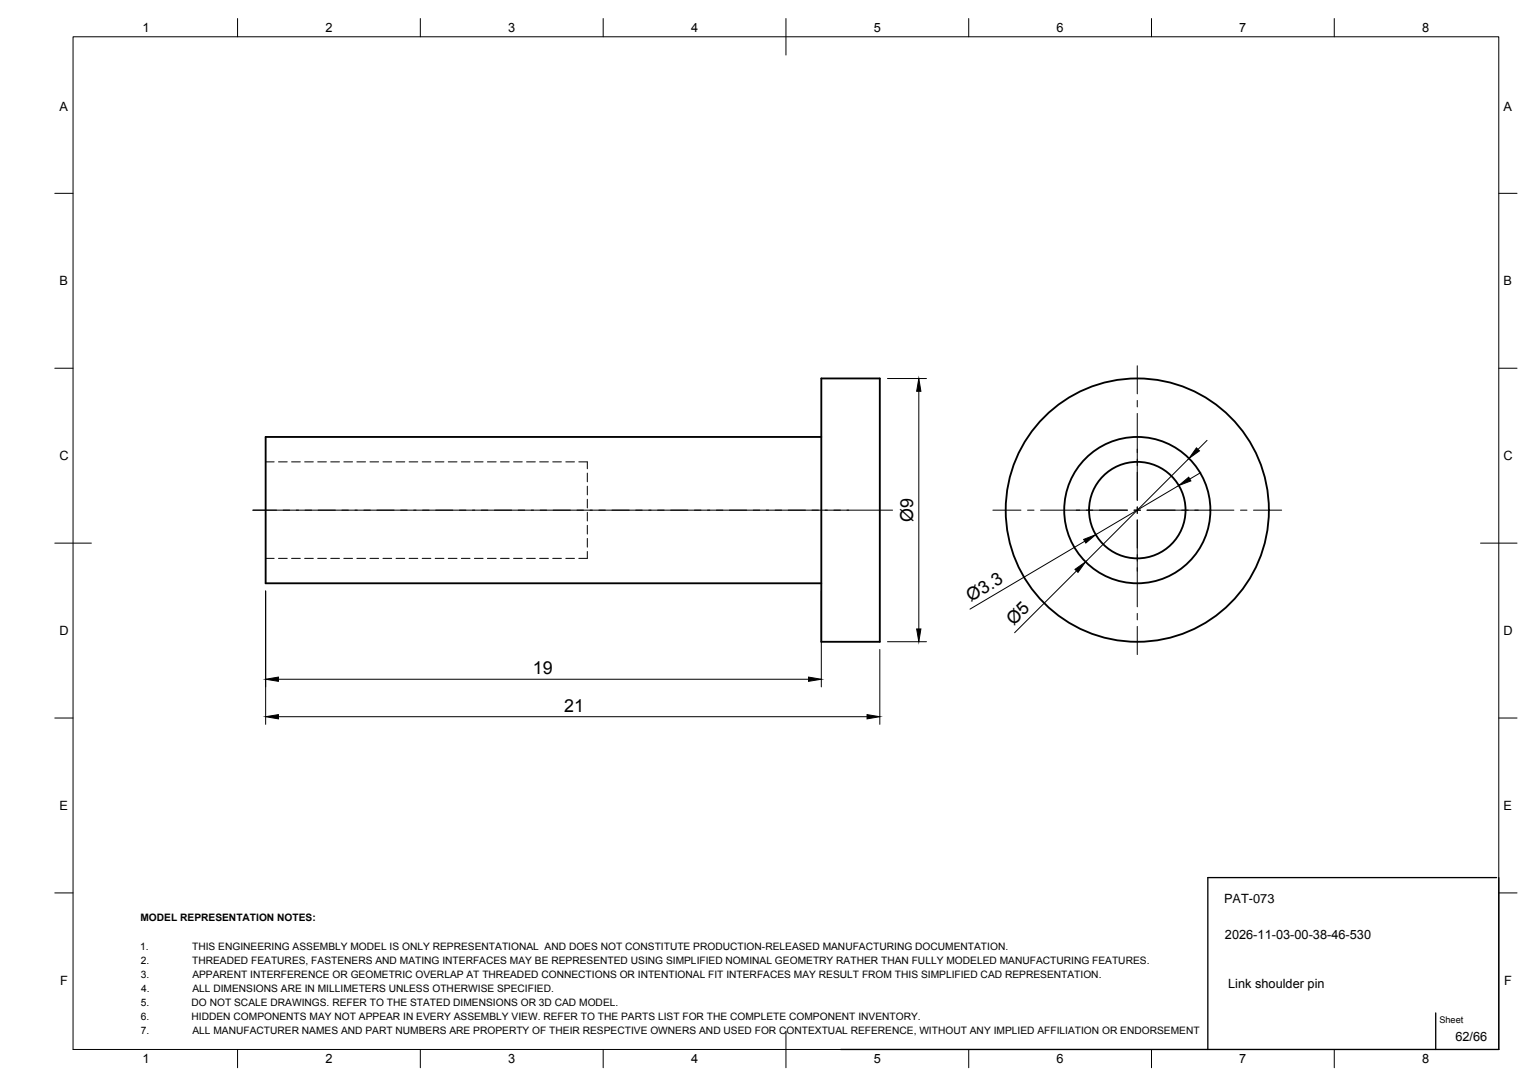
ISO-10303-21;
HEADER;
/* Generated by software containing ST-Developer
 * from STEP Tools, Inc. (www.steptools.com) 
 */

FILE_DESCRIPTION(
/* description */ ('Manual piston pump'),
/* implementation_level */ '2;1');

FILE_NAME(
/* name */ 'Link shoulder pin.step',
/* time_stamp */ '2026-11-02T16:54:23-08:00',
/* author */ (''),
/* organization */ (''),
/* preprocessor_version */ 'ST-DEVELOPER v20.2',
/* originating_system */ 'Autodesk Translation Framework v15.17.0.0',
/* authorisation */ '');

FILE_SCHEMA (('AUTOMOTIVE_DESIGN { 1 0 10303 214 3 1 1 }'));
ENDSEC;

DATA;
#10=MECHANICAL_DESIGN_GEOMETRIC_PRESENTATION_REPRESENTATION('',(#754),#19043);
#619=SHAPE_REPRESENTATION_RELATIONSHIP('SRR','None',#19369,#682);
#682=ADVANCED_BREP_SHAPE_REPRESENTATION('',(#822),#19036);
#754=STYLED_ITEM('',(#19661),#822);
#822=MANIFOLD_SOLID_BREP('Body1',#9542);
#1035=FACE_BOUND('',#2610,.T.);
#1036=FACE_BOUND('',#2615,.T.);
#1277=CYLINDRICAL_SURFACE('',#11382,0.164999999999999);
#1278=CYLINDRICAL_SURFACE('',#11389,0.449999999999999);
#1279=CYLINDRICAL_SURFACE('',#11392,0.25);
#1824=FACE_OUTER_BOUND('',#2607,.T.);
#1825=FACE_OUTER_BOUND('',#2608,.T.);
#1826=FACE_OUTER_BOUND('',#2609,.T.);
#1827=FACE_OUTER_BOUND('',#2611,.T.);
#1828=FACE_OUTER_BOUND('',#2612,.T.);
#1829=FACE_OUTER_BOUND('',#2613,.T.);
#1830=FACE_OUTER_BOUND('',#2614,.T.);
#2607=EDGE_LOOP('',(#8423,#8424,#8425,#8426));
#2608=EDGE_LOOP('',(#8427));
#2609=EDGE_LOOP('',(#8428));
#2610=EDGE_LOOP('',(#8429));
#2611=EDGE_LOOP('',(#8430,#8431,#8432,#8433));
#2612=EDGE_LOOP('',(#8434));
#2613=EDGE_LOOP('',(#8435,#8436,#8437,#8438));
#2614=EDGE_LOOP('',(#8439));
#2615=EDGE_LOOP('',(#8440));
#3114=CIRCLE('',#11383,0.164999999999999);
#3115=CIRCLE('',#11384,0.164999999999999);
#3116=CIRCLE('',#11387,0.449999999999999);
#3117=CIRCLE('',#11388,0.25);
#3118=CIRCLE('',#11390,0.449999999999999);
#3119=CIRCLE('',#11393,0.25);
#3709=LINE('',#18702,#4313);
#3710=LINE('',#18712,#4314);
#3711=LINE('',#18718,#4315);
#4313=VECTOR('',#14339,0.164999999999999);
#4314=VECTOR('',#14352,0.449999999999999);
#4315=VECTOR('',#14361,0.25);
#5074=VERTEX_POINT('',#18699);
#5075=VERTEX_POINT('',#18701);
#5076=VERTEX_POINT('',#18706);
#5077=VERTEX_POINT('',#18708);
#5078=VERTEX_POINT('',#18711);
#5079=VERTEX_POINT('',#18716);
#6198=EDGE_CURVE('',#5074,#5074,#3114,.T.);
#6199=EDGE_CURVE('',#5074,#5075,#3709,.T.);
#6200=EDGE_CURVE('',#5075,#5075,#3115,.T.);
#6201=EDGE_CURVE('',#5076,#5076,#3116,.T.);
#6202=EDGE_CURVE('',#5077,#5077,#3117,.T.);
#6203=EDGE_CURVE('',#5076,#5078,#3710,.T.);
#6204=EDGE_CURVE('',#5078,#5078,#3118,.T.);
#6205=EDGE_CURVE('',#5079,#5079,#3119,.T.);
#6206=EDGE_CURVE('',#5079,#5077,#3711,.T.);
#8423=ORIENTED_EDGE('',*,*,#6198,.F.);
#8424=ORIENTED_EDGE('',*,*,#6199,.T.);
#8425=ORIENTED_EDGE('',*,*,#6200,.F.);
#8426=ORIENTED_EDGE('',*,*,#6199,.F.);
#8427=ORIENTED_EDGE('',*,*,#6198,.T.);
#8428=ORIENTED_EDGE('',*,*,#6201,.T.);
#8429=ORIENTED_EDGE('',*,*,#6202,.F.);
#8430=ORIENTED_EDGE('',*,*,#6201,.F.);
#8431=ORIENTED_EDGE('',*,*,#6203,.T.);
#8432=ORIENTED_EDGE('',*,*,#6204,.T.);
#8433=ORIENTED_EDGE('',*,*,#6203,.F.);
#8434=ORIENTED_EDGE('',*,*,#6204,.F.);
#8435=ORIENTED_EDGE('',*,*,#6205,.F.);
#8436=ORIENTED_EDGE('',*,*,#6206,.T.);
#8437=ORIENTED_EDGE('',*,*,#6202,.T.);
#8438=ORIENTED_EDGE('',*,*,#6206,.F.);
#8439=ORIENTED_EDGE('',*,*,#6205,.T.);
#8440=ORIENTED_EDGE('',*,*,#6200,.T.);
#8872=PLANE('',#11385);
#8873=PLANE('',#11386);
#8874=PLANE('',#11391);
#8875=PLANE('',#11394);
#9429=ADVANCED_FACE('',(#1824),#1277,.F.);
#9430=ADVANCED_FACE('',(#1825),#8872,.T.);
#9431=ADVANCED_FACE('',(#1826,#1035),#8873,.T.);
#9432=ADVANCED_FACE('',(#1827),#1278,.T.);
#9433=ADVANCED_FACE('',(#1828),#8874,.F.);
#9434=ADVANCED_FACE('',(#1829),#1279,.T.);
#9435=ADVANCED_FACE('',(#1830,#1036),#8875,.T.);
#9542=CLOSED_SHELL('',(#9429,#9430,#9431,#9432,#9433,#9434,#9435));
#11381=AXIS2_PLACEMENT_3D('',#18697,#14333,#14334);
#11382=AXIS2_PLACEMENT_3D('',#18698,#14335,#14336);
#11383=AXIS2_PLACEMENT_3D('',#18700,#14337,#14338);
#11384=AXIS2_PLACEMENT_3D('',#18703,#14340,#14341);
#11385=AXIS2_PLACEMENT_3D('',#18704,#14342,#14343);
#11386=AXIS2_PLACEMENT_3D('',#18705,#14344,#14345);
#11387=AXIS2_PLACEMENT_3D('',#18707,#14346,#14347);
#11388=AXIS2_PLACEMENT_3D('',#18709,#14348,#14349);
#11389=AXIS2_PLACEMENT_3D('',#18710,#14350,#14351);
#11390=AXIS2_PLACEMENT_3D('',#18713,#14353,#14354);
#11391=AXIS2_PLACEMENT_3D('',#18714,#14355,#14356);
#11392=AXIS2_PLACEMENT_3D('',#18715,#14357,#14358);
#11393=AXIS2_PLACEMENT_3D('',#18717,#14359,#14360);
#11394=AXIS2_PLACEMENT_3D('',#18719,#14362,#14363);
#14333=DIRECTION('axis',(0.,0.,1.));
#14334=DIRECTION('refdir',(1.,0.,0.));
#14335=DIRECTION('center_axis',(1.,0.,0.));
#14336=DIRECTION('ref_axis',(0.,0.,-1.));
#14337=DIRECTION('center_axis',(1.,0.,0.));
#14338=DIRECTION('ref_axis',(0.,0.,-1.));
#14339=DIRECTION('',(1.,0.,0.));
#14340=DIRECTION('center_axis',(-1.,0.,0.));
#14341=DIRECTION('ref_axis',(0.,0.,-1.));
#14342=DIRECTION('center_axis',(1.,0.,0.));
#14343=DIRECTION('ref_axis',(0.,0.,-1.));
#14344=DIRECTION('center_axis',(1.,0.,0.));
#14345=DIRECTION('ref_axis',(0.,0.,-1.));
#14346=DIRECTION('center_axis',(1.,0.,0.));
#14347=DIRECTION('ref_axis',(0.,0.,-1.));
#14348=DIRECTION('center_axis',(1.,0.,0.));
#14349=DIRECTION('ref_axis',(0.,0.,-1.));
#14350=DIRECTION('center_axis',(1.,0.,0.));
#14351=DIRECTION('ref_axis',(0.,0.,-1.));
#14352=DIRECTION('',(-1.,0.,0.));
#14353=DIRECTION('center_axis',(1.,0.,0.));
#14354=DIRECTION('ref_axis',(0.,0.,-1.));
#14355=DIRECTION('center_axis',(1.,0.,0.));
#14356=DIRECTION('ref_axis',(0.,0.,-1.));
#14357=DIRECTION('center_axis',(1.,0.,0.));
#14358=DIRECTION('ref_axis',(0.,0.,-1.));
#14359=DIRECTION('center_axis',(1.,0.,0.));
#14360=DIRECTION('ref_axis',(0.,0.,-1.));
#14361=DIRECTION('',(-1.,0.,0.));
#14362=DIRECTION('center_axis',(1.,0.,0.));
#14363=DIRECTION('ref_axis',(0.,0.,-1.));
#18697=CARTESIAN_POINT('',(0.,0.,0.));
#18698=CARTESIAN_POINT('Origin',(-0.6,-8.,10.));
#18699=CARTESIAN_POINT('',(-0.6,-8.,10.165));
#18700=CARTESIAN_POINT('Origin',(-0.6,-8.,10.));
#18701=CARTESIAN_POINT('',(0.5,-8.,10.165));
#18702=CARTESIAN_POINT('',(-0.6,-8.,10.165));
#18703=CARTESIAN_POINT('Origin',(0.5,-8.,10.));
#18704=CARTESIAN_POINT('Origin',(-0.6,-8.,10.));
#18705=CARTESIAN_POINT('Origin',(-1.4,-8.,10.));
#18706=CARTESIAN_POINT('',(-1.4,-8.,10.45));
#18707=CARTESIAN_POINT('Origin',(-1.4,-8.,10.));
#18708=CARTESIAN_POINT('',(-1.4,-8.,10.25));
#18709=CARTESIAN_POINT('Origin',(-1.4,-8.,10.));
#18710=CARTESIAN_POINT('Origin',(-1.6,-8.,10.));
#18711=CARTESIAN_POINT('',(-1.6,-8.,10.45));
#18712=CARTESIAN_POINT('',(-1.6,-8.,10.45));
#18713=CARTESIAN_POINT('Origin',(-1.6,-8.,10.));
#18714=CARTESIAN_POINT('Origin',(-1.6,-8.,10.));
#18715=CARTESIAN_POINT('Origin',(-1.4,-8.,10.));
#18716=CARTESIAN_POINT('',(0.5,-8.,10.25));
#18717=CARTESIAN_POINT('Origin',(0.5,-8.,10.));
#18718=CARTESIAN_POINT('',(-1.4,-8.,10.25));
#18719=CARTESIAN_POINT('Origin',(0.5,-8.,10.));
#18965=UNCERTAINTY_MEASURE_WITH_UNIT(LENGTH_MEASURE(0.001),#19044,
'DISTANCE_ACCURACY_VALUE',
'Maximum model space distance between geometric entities at asserted c
onnectivities');
#18972=UNCERTAINTY_MEASURE_WITH_UNIT(LENGTH_MEASURE(0.001),#19044,
'DISTANCE_ACCURACY_VALUE',
'Maximum model space distance between geometric entities at asserted c
onnectivities');
#19036=(
GEOMETRIC_REPRESENTATION_CONTEXT(3)
GLOBAL_UNCERTAINTY_ASSIGNED_CONTEXT((#18965))
GLOBAL_UNIT_ASSIGNED_CONTEXT((#19044,#19046,#19047))
REPRESENTATION_CONTEXT('','3D')
);
#19043=(
GEOMETRIC_REPRESENTATION_CONTEXT(3)
GLOBAL_UNCERTAINTY_ASSIGNED_CONTEXT((#18972))
GLOBAL_UNIT_ASSIGNED_CONTEXT((#19044,#19046,#19047))
REPRESENTATION_CONTEXT('','3D')
);
#19044=(
LENGTH_UNIT()
NAMED_UNIT(*)
SI_UNIT(.CENTI.,.METRE.)
);
#19046=(
NAMED_UNIT(*)
PLANE_ANGLE_UNIT()
SI_UNIT($,.RADIAN.)
);
#19047=(
NAMED_UNIT(*)
SI_UNIT($,.STERADIAN.)
SOLID_ANGLE_UNIT()
);
#19111=SHAPE_DEFINITION_REPRESENTATION(#19268,#19369);
#19268=PRODUCT_DEFINITION_SHAPE('',$,#19440);
#19369=SHAPE_REPRESENTATION('',(#11381),#19036);
#19376=PRODUCT_DEFINITION_CONTEXT('part definition',#19588,'design');
#19440=PRODUCT_DEFINITION('2026-11-03-00-38-46-530','Link shoulder pin',
#19510,#19376);
#19510=PRODUCT_DEFINITION_FORMATION('',$,#19653);
#19588=APPLICATION_CONTEXT(
'Core Data for Automotive Mechanical Design Process');
#19589=PRODUCT_CONTEXT('part definition',#19588,'mechanical');
#19653=PRODUCT('2026-11-03-00-38-46-530','Link shoulder pin',
'Link shoulder pin',(#19589));
#19661=PRESENTATION_STYLE_ASSIGNMENT((#19667));
#19667=SURFACE_STYLE_USAGE(.BOTH.,#19673);
#19673=SURFACE_SIDE_STYLE('',(#19679));
#19679=SURFACE_STYLE_FILL_AREA(#19685);
#19685=FILL_AREA_STYLE('CAD Library Painted - Engineering blue',(#19691));
#19691=FILL_AREA_STYLE_COLOUR('CAD Library Painted - Engineering blue',
#19697);
#19697=COLOUR_RGB('CAD Library Painted - Engineering blue',0.12156862745098,
0.356862745098039,0.6);
ENDSEC;
END-ISO-10303-21;
